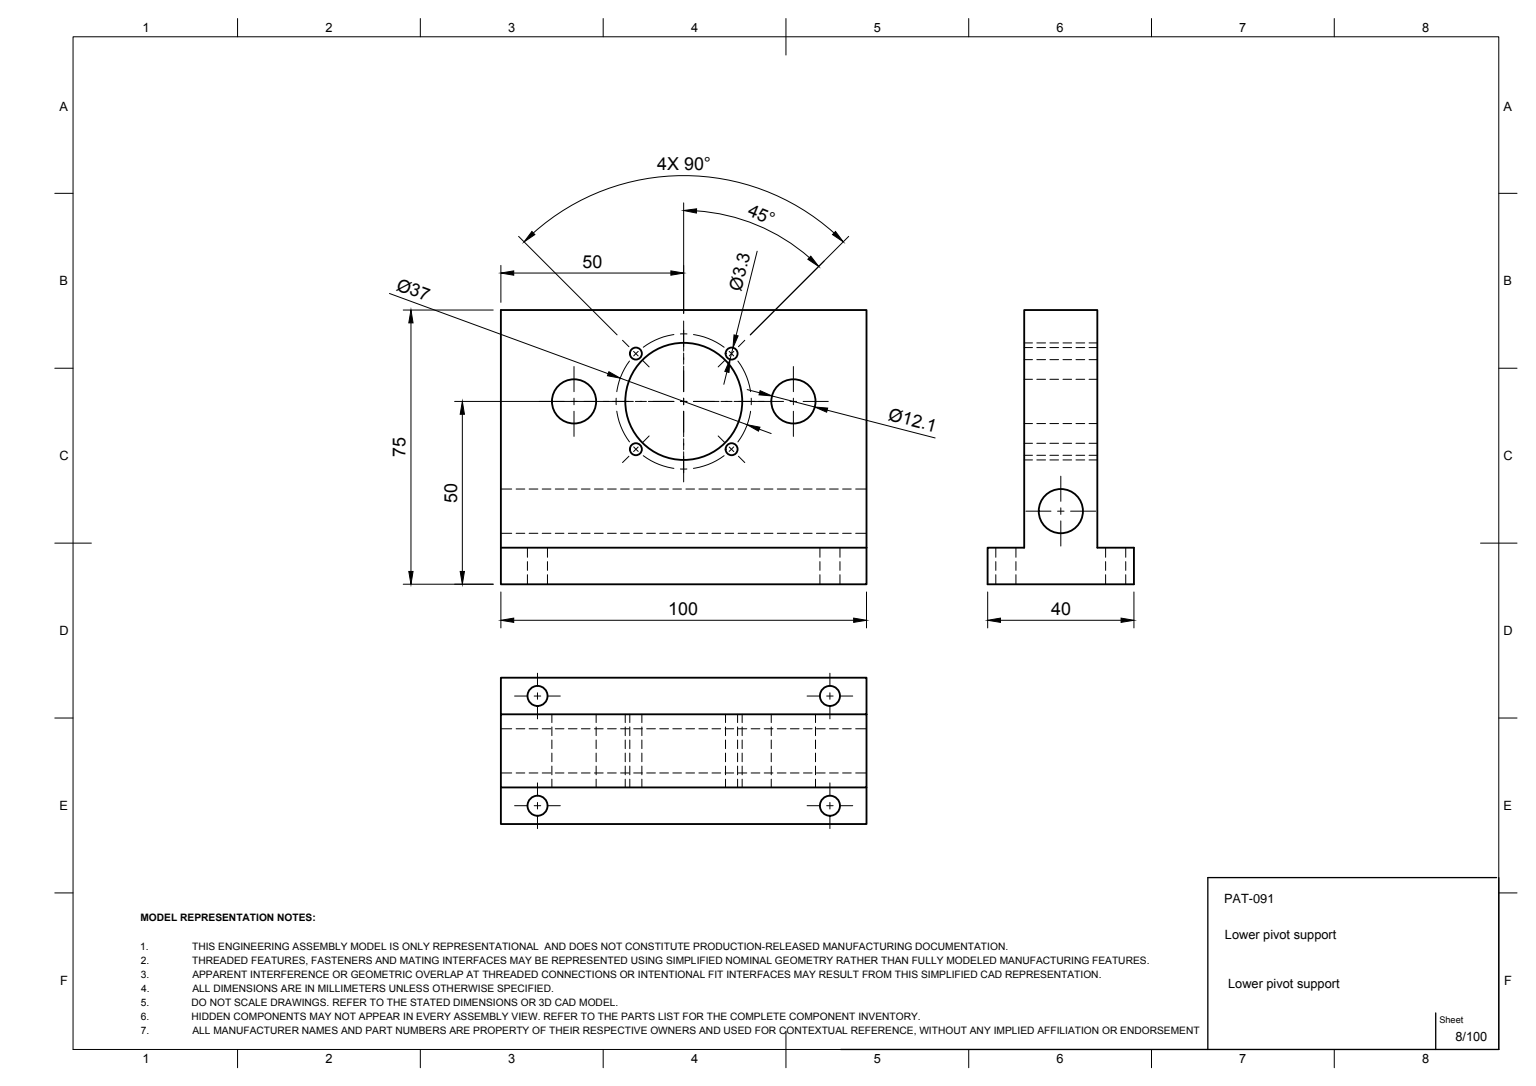
ISO-10303-21;
HEADER;
/* Generated by software containing ST-Developer
 * from STEP Tools, Inc. (www.steptools.com) 
 */

FILE_DESCRIPTION(
/* description */ ('PAT-091'),
/* implementation_level */ '2;1');

FILE_NAME(
/* name */ 'Lower pivot support.step',
/* time_stamp */ '2026-10-27T15:34:44-07:00',
/* author */ (''),
/* organization */ (''),
/* preprocessor_version */ 'ST-DEVELOPER v20.2',
/* originating_system */ 'Autodesk Translation Framework v15.17.0.0',
/* authorisation */ '');

FILE_SCHEMA (('AUTOMOTIVE_DESIGN { 1 0 10303 214 3 1 1 }'));
ENDSEC;

DATA;
#10=MECHANICAL_DESIGN_GEOMETRIC_PRESENTATION_REPRESENTATION('',(#974),#25100);
#754=SHAPE_REPRESENTATION_RELATIONSHIP('SRR','None',#25515,#864);
#864=ADVANCED_BREP_SHAPE_REPRESENTATION('',(#1098),#24985);
#974=STYLED_ITEM('',(#26177),#1098);
#1098=MANIFOLD_SOLID_BREP('Body1',#13251);
#1231=FACE_BOUND('',#2933,.T.);
#1232=FACE_BOUND('',#2934,.T.);
#1233=FACE_BOUND('',#2936,.T.);
#1234=FACE_BOUND('',#2937,.T.);
#1235=FACE_BOUND('',#2941,.T.);
#1236=FACE_BOUND('',#2943,.T.);
#1237=FACE_BOUND('',#2944,.T.);
#1238=FACE_BOUND('',#2945,.T.);
#1239=FACE_BOUND('',#2946,.T.);
#1240=FACE_BOUND('',#2947,.T.);
#1241=FACE_BOUND('',#2948,.T.);
#1242=FACE_BOUND('',#2949,.T.);
#1243=FACE_BOUND('',#2954,.T.);
#1244=FACE_BOUND('',#2955,.T.);
#1245=FACE_BOUND('',#2956,.T.);
#1246=FACE_BOUND('',#2957,.T.);
#1247=FACE_BOUND('',#2958,.T.);
#1248=FACE_BOUND('',#2959,.T.);
#1249=FACE_BOUND('',#2960,.T.);
#1250=FACE_BOUND('',#2962,.T.);
#1251=FACE_BOUND('',#2965,.T.);
#1252=FACE_BOUND('',#2966,.T.);
#1253=FACE_BOUND('',#2967,.T.);
#1254=FACE_BOUND('',#2968,.T.);
#1658=PLANE('',#14660);
#1659=PLANE('',#14661);
#1660=PLANE('',#14662);
#1661=PLANE('',#14663);
#1662=PLANE('',#14664);
#1663=PLANE('',#14666);
#1664=PLANE('',#14675);
#1665=PLANE('',#14676);
#1666=PLANE('',#14677);
#1667=PLANE('',#14678);
#2089=FACE_OUTER_BOUND('',#2923,.T.);
#2090=FACE_OUTER_BOUND('',#2924,.T.);
#2091=FACE_OUTER_BOUND('',#2925,.T.);
#2092=FACE_OUTER_BOUND('',#2926,.T.);
#2093=FACE_OUTER_BOUND('',#2927,.T.);
#2094=FACE_OUTER_BOUND('',#2928,.T.);
#2095=FACE_OUTER_BOUND('',#2929,.T.);
#2096=FACE_OUTER_BOUND('',#2930,.T.);
#2097=FACE_OUTER_BOUND('',#2931,.T.);
#2098=FACE_OUTER_BOUND('',#2932,.T.);
#2099=FACE_OUTER_BOUND('',#2935,.T.);
#2100=FACE_OUTER_BOUND('',#2938,.T.);
#2101=FACE_OUTER_BOUND('',#2939,.T.);
#2102=FACE_OUTER_BOUND('',#2940,.T.);
#2103=FACE_OUTER_BOUND('',#2942,.T.);
#2104=FACE_OUTER_BOUND('',#2950,.T.);
#2105=FACE_OUTER_BOUND('',#2951,.T.);
#2106=FACE_OUTER_BOUND('',#2952,.T.);
#2107=FACE_OUTER_BOUND('',#2953,.T.);
#2108=FACE_OUTER_BOUND('',#2961,.T.);
#2109=FACE_OUTER_BOUND('',#2963,.T.);
#2110=FACE_OUTER_BOUND('',#2964,.T.);
#2923=EDGE_LOOP('',(#9092,#9093,#9094,#9095));
#2924=EDGE_LOOP('',(#9096,#9097,#9098,#9099));
#2925=EDGE_LOOP('',(#9100,#9101,#9102,#9103));
#2926=EDGE_LOOP('',(#9104,#9105,#9106,#9107));
#2927=EDGE_LOOP('',(#9108,#9109,#9110,#9111));
#2928=EDGE_LOOP('',(#9112,#9113,#9114,#9115));
#2929=EDGE_LOOP('',(#9116,#9117,#9118,#9119));
#2930=EDGE_LOOP('',(#9120,#9121,#9122,#9123));
#2931=EDGE_LOOP('',(#9124,#9125,#9126,#9127));
#2932=EDGE_LOOP('',(#9128,#9129,#9130,#9131));
#2933=EDGE_LOOP('',(#9132));
#2934=EDGE_LOOP('',(#9133));
#2935=EDGE_LOOP('',(#9134,#9135,#9136,#9137));
#2936=EDGE_LOOP('',(#9138));
#2937=EDGE_LOOP('',(#9139));
#2938=EDGE_LOOP('',(#9140,#9141,#9142,#9143));
#2939=EDGE_LOOP('',(#9144,#9145,#9146,#9147));
#2940=EDGE_LOOP('',(#9148,#9149,#9150,#9151,#9152,#9153,#9154,#9155));
#2941=EDGE_LOOP('',(#9156));
#2942=EDGE_LOOP('',(#9157,#9158,#9159,#9160));
#2943=EDGE_LOOP('',(#9161));
#2944=EDGE_LOOP('',(#9162));
#2945=EDGE_LOOP('',(#9163));
#2946=EDGE_LOOP('',(#9164));
#2947=EDGE_LOOP('',(#9165));
#2948=EDGE_LOOP('',(#9166));
#2949=EDGE_LOOP('',(#9167));
#2950=EDGE_LOOP('',(#9168,#9169,#9170,#9171));
#2951=EDGE_LOOP('',(#9172,#9173,#9174,#9175));
#2952=EDGE_LOOP('',(#9176,#9177,#9178,#9179));
#2953=EDGE_LOOP('',(#9180,#9181,#9182,#9183));
#2954=EDGE_LOOP('',(#9184));
#2955=EDGE_LOOP('',(#9185));
#2956=EDGE_LOOP('',(#9186));
#2957=EDGE_LOOP('',(#9187));
#2958=EDGE_LOOP('',(#9188));
#2959=EDGE_LOOP('',(#9189));
#2960=EDGE_LOOP('',(#9190));
#2961=EDGE_LOOP('',(#9191,#9192,#9193,#9194,#9195,#9196,#9197,#9198));
#2962=EDGE_LOOP('',(#9199));
#2963=EDGE_LOOP('',(#9200,#9201,#9202,#9203));
#2964=EDGE_LOOP('',(#9204,#9205,#9206,#9207));
#2965=EDGE_LOOP('',(#9208));
#2966=EDGE_LOOP('',(#9209));
#2967=EDGE_LOOP('',(#9210));
#2968=EDGE_LOOP('',(#9211));
#4168=LINE('',#21110,#4908);
#4169=LINE('',#21116,#4909);
#4170=LINE('',#21122,#4910);
#4171=LINE('',#21128,#4911);
#4172=LINE('',#21134,#4912);
#4173=LINE('',#21140,#4913);
#4174=LINE('',#21146,#4914);
#4175=LINE('',#21152,#4915);
#4176=LINE('',#21158,#4916);
#4177=LINE('',#21163,#4917);
#4178=LINE('',#21165,#4918);
#4179=LINE('',#21167,#4919);
#4180=LINE('',#21168,#4920);
#4181=LINE('',#21172,#4921);
#4182=LINE('',#21174,#4922);
#4183=LINE('',#21176,#4923);
#4184=LINE('',#21177,#4924);
#4185=LINE('',#21181,#4925);
#4186=LINE('',#21182,#4926);
#4187=LINE('',#21183,#4927);
#4188=LINE('',#21187,#4928);
#4189=LINE('',#21188,#4929);
#4190=LINE('',#21189,#4930);
#4191=LINE('',#21192,#4931);
#4192=LINE('',#21194,#4932);
#4193=LINE('',#21195,#4933);
#4194=LINE('',#21196,#4934);
#4195=LINE('',#21201,#4935);
#4196=LINE('',#21202,#4936);
#4197=LINE('',#21210,#4937);
#4198=LINE('',#21213,#4938);
#4199=LINE('',#21217,#4939);
#4200=LINE('',#21221,#4940);
#4201=LINE('',#21222,#4941);
#4202=LINE('',#21224,#4942);
#4203=LINE('',#21225,#4943);
#4908=VECTOR('',#16612,0.165);
#4909=VECTOR('',#16619,0.165);
#4910=VECTOR('',#16626,0.165);
#4911=VECTOR('',#16633,0.165);
#4912=VECTOR('',#16640,1.6);
#4913=VECTOR('',#16647,0.275);
#4914=VECTOR('',#16654,0.275);
#4915=VECTOR('',#16661,0.275);
#4916=VECTOR('',#16668,0.275);
#4917=VECTOR('',#16673,1.);
#4918=VECTOR('',#16674,1.);
#4919=VECTOR('',#16675,1.);
#4920=VECTOR('',#16676,1.);
#4921=VECTOR('',#16679,1.);
#4922=VECTOR('',#16680,1.);
#4923=VECTOR('',#16681,1.);
#4924=VECTOR('',#16682,1.);
#4925=VECTOR('',#16685,1.);
#4926=VECTOR('',#16686,1.);
#4927=VECTOR('',#16687,1.);
#4928=VECTOR('',#16690,1.);
#4929=VECTOR('',#16691,1.);
#4930=VECTOR('',#16692,1.);
#4931=VECTOR('',#16695,1.);
#4932=VECTOR('',#16696,1.);
#4933=VECTOR('',#16697,1.);
#4934=VECTOR('',#16698,1.);
#4935=VECTOR('',#16703,1.);
#4936=VECTOR('',#16704,1.);
#4937=VECTOR('',#16713,0.605);
#4938=VECTOR('',#16716,0.605);
#4939=VECTOR('',#16721,0.605);
#4940=VECTOR('',#16726,1.);
#4941=VECTOR('',#16727,1.);
#4942=VECTOR('',#16730,1.);
#4943=VECTOR('',#16731,1.);
#5620=CIRCLE('',#14634,0.165);
#5621=CIRCLE('',#14635,0.165);
#5622=CIRCLE('',#14637,0.165);
#5623=CIRCLE('',#14638,0.165);
#5624=CIRCLE('',#14640,0.165);
#5625=CIRCLE('',#14641,0.165);
#5626=CIRCLE('',#14643,0.165);
#5627=CIRCLE('',#14644,0.165);
#5628=CIRCLE('',#14646,1.6);
#5629=CIRCLE('',#14647,1.6);
#5630=CIRCLE('',#14649,0.275);
#5631=CIRCLE('',#14650,0.275);
#5632=CIRCLE('',#14652,0.275);
#5633=CIRCLE('',#14653,0.275);
#5634=CIRCLE('',#14655,0.275);
#5635=CIRCLE('',#14656,0.275);
#5636=CIRCLE('',#14658,0.275);
#5637=CIRCLE('',#14659,0.275);
#5638=CIRCLE('',#14665,0.605);
#5639=CIRCLE('',#14667,0.605);
#5640=CIRCLE('',#14668,0.605);
#5641=CIRCLE('',#14670,0.605);
#5642=CIRCLE('',#14672,0.605);
#5643=CIRCLE('',#14674,0.605);
#6423=VERTEX_POINT('',#21107);
#6424=VERTEX_POINT('',#21109);
#6425=VERTEX_POINT('',#21113);
#6426=VERTEX_POINT('',#21115);
#6427=VERTEX_POINT('',#21119);
#6428=VERTEX_POINT('',#21121);
#6429=VERTEX_POINT('',#21125);
#6430=VERTEX_POINT('',#21127);
#6431=VERTEX_POINT('',#21131);
#6432=VERTEX_POINT('',#21133);
#6433=VERTEX_POINT('',#21137);
#6434=VERTEX_POINT('',#21139);
#6435=VERTEX_POINT('',#21143);
#6436=VERTEX_POINT('',#21145);
#6437=VERTEX_POINT('',#21149);
#6438=VERTEX_POINT('',#21151);
#6439=VERTEX_POINT('',#21155);
#6440=VERTEX_POINT('',#21157);
#6441=VERTEX_POINT('',#21161);
#6442=VERTEX_POINT('',#21162);
#6443=VERTEX_POINT('',#21164);
#6444=VERTEX_POINT('',#21166);
#6445=VERTEX_POINT('',#21170);
#6446=VERTEX_POINT('',#21171);
#6447=VERTEX_POINT('',#21173);
#6448=VERTEX_POINT('',#21175);
#6449=VERTEX_POINT('',#21179);
#6450=VERTEX_POINT('',#21180);
#6451=VERTEX_POINT('',#21185);
#6452=VERTEX_POINT('',#21186);
#6453=VERTEX_POINT('',#21191);
#6454=VERTEX_POINT('',#21193);
#6455=VERTEX_POINT('',#21197);
#6456=VERTEX_POINT('',#21200);
#6457=VERTEX_POINT('',#21203);
#6458=VERTEX_POINT('',#21205);
#6459=VERTEX_POINT('',#21208);
#6460=VERTEX_POINT('',#21212);
#6461=VERTEX_POINT('',#21216);
#6462=VERTEX_POINT('',#21220);
#7481=EDGE_CURVE('',#6423,#6423,#5620,.T.);
#7482=EDGE_CURVE('',#6423,#6424,#4168,.T.);
#7483=EDGE_CURVE('',#6424,#6424,#5621,.T.);
#7484=EDGE_CURVE('',#6425,#6425,#5622,.T.);
#7485=EDGE_CURVE('',#6425,#6426,#4169,.T.);
#7486=EDGE_CURVE('',#6426,#6426,#5623,.T.);
#7487=EDGE_CURVE('',#6427,#6427,#5624,.T.);
#7488=EDGE_CURVE('',#6427,#6428,#4170,.T.);
#7489=EDGE_CURVE('',#6428,#6428,#5625,.T.);
#7490=EDGE_CURVE('',#6429,#6429,#5626,.T.);
#7491=EDGE_CURVE('',#6429,#6430,#4171,.T.);
#7492=EDGE_CURVE('',#6430,#6430,#5627,.T.);
#7493=EDGE_CURVE('',#6431,#6431,#5628,.T.);
#7494=EDGE_CURVE('',#6431,#6432,#4172,.T.);
#7495=EDGE_CURVE('',#6432,#6432,#5629,.T.);
#7496=EDGE_CURVE('',#6433,#6433,#5630,.T.);
#7497=EDGE_CURVE('',#6433,#6434,#4173,.T.);
#7498=EDGE_CURVE('',#6434,#6434,#5631,.T.);
#7499=EDGE_CURVE('',#6435,#6435,#5632,.T.);
#7500=EDGE_CURVE('',#6435,#6436,#4174,.T.);
#7501=EDGE_CURVE('',#6436,#6436,#5633,.T.);
#7502=EDGE_CURVE('',#6437,#6437,#5634,.T.);
#7503=EDGE_CURVE('',#6437,#6438,#4175,.T.);
#7504=EDGE_CURVE('',#6438,#6438,#5635,.T.);
#7505=EDGE_CURVE('',#6439,#6439,#5636,.T.);
#7506=EDGE_CURVE('',#6439,#6440,#4176,.T.);
#7507=EDGE_CURVE('',#6440,#6440,#5637,.T.);
#7508=EDGE_CURVE('',#6441,#6442,#4177,.T.);
#7509=EDGE_CURVE('',#6441,#6443,#4178,.T.);
#7510=EDGE_CURVE('',#6443,#6444,#4179,.T.);
#7511=EDGE_CURVE('',#6444,#6442,#4180,.T.);
#7512=EDGE_CURVE('',#6445,#6446,#4181,.T.);
#7513=EDGE_CURVE('',#6445,#6447,#4182,.T.);
#7514=EDGE_CURVE('',#6447,#6448,#4183,.T.);
#7515=EDGE_CURVE('',#6448,#6446,#4184,.T.);
#7516=EDGE_CURVE('',#6449,#6450,#4185,.T.);
#7517=EDGE_CURVE('',#6450,#6448,#4186,.T.);
#7518=EDGE_CURVE('',#6449,#6447,#4187,.T.);
#7519=EDGE_CURVE('',#6451,#6452,#4188,.T.);
#7520=EDGE_CURVE('',#6452,#6444,#4189,.T.);
#7521=EDGE_CURVE('',#6451,#6443,#4190,.T.);
#7522=EDGE_CURVE('',#6441,#6453,#4191,.T.);
#7523=EDGE_CURVE('',#6454,#6453,#4192,.T.);
#7524=EDGE_CURVE('',#6446,#6454,#4193,.T.);
#7525=EDGE_CURVE('',#6450,#6451,#4194,.T.);
#7526=EDGE_CURVE('',#6455,#6455,#5638,.T.);
#7527=EDGE_CURVE('',#6442,#6456,#4195,.T.);
#7528=EDGE_CURVE('',#6453,#6456,#4196,.T.);
#7529=EDGE_CURVE('',#6457,#6457,#5639,.T.);
#7530=EDGE_CURVE('',#6458,#6458,#5640,.T.);
#7531=EDGE_CURVE('',#6459,#6459,#5641,.T.);
#7532=EDGE_CURVE('',#6459,#6455,#4197,.T.);
#7533=EDGE_CURVE('',#6457,#6460,#4198,.T.);
#7534=EDGE_CURVE('',#6460,#6460,#5642,.T.);
#7535=EDGE_CURVE('',#6458,#6461,#4199,.T.);
#7536=EDGE_CURVE('',#6461,#6461,#5643,.T.);
#7537=EDGE_CURVE('',#6462,#6454,#4200,.T.);
#7538=EDGE_CURVE('',#6445,#6462,#4201,.T.);
#7539=EDGE_CURVE('',#6456,#6462,#4202,.T.);
#7540=EDGE_CURVE('',#6452,#6449,#4203,.T.);
#9092=ORIENTED_EDGE('',*,*,#7481,.F.);
#9093=ORIENTED_EDGE('',*,*,#7482,.T.);
#9094=ORIENTED_EDGE('',*,*,#7483,.F.);
#9095=ORIENTED_EDGE('',*,*,#7482,.F.);
#9096=ORIENTED_EDGE('',*,*,#7484,.F.);
#9097=ORIENTED_EDGE('',*,*,#7485,.T.);
#9098=ORIENTED_EDGE('',*,*,#7486,.F.);
#9099=ORIENTED_EDGE('',*,*,#7485,.F.);
#9100=ORIENTED_EDGE('',*,*,#7487,.F.);
#9101=ORIENTED_EDGE('',*,*,#7488,.T.);
#9102=ORIENTED_EDGE('',*,*,#7489,.F.);
#9103=ORIENTED_EDGE('',*,*,#7488,.F.);
#9104=ORIENTED_EDGE('',*,*,#7490,.F.);
#9105=ORIENTED_EDGE('',*,*,#7491,.T.);
#9106=ORIENTED_EDGE('',*,*,#7492,.F.);
#9107=ORIENTED_EDGE('',*,*,#7491,.F.);
#9108=ORIENTED_EDGE('',*,*,#7493,.F.);
#9109=ORIENTED_EDGE('',*,*,#7494,.T.);
#9110=ORIENTED_EDGE('',*,*,#7495,.F.);
#9111=ORIENTED_EDGE('',*,*,#7494,.F.);
#9112=ORIENTED_EDGE('',*,*,#7496,.F.);
#9113=ORIENTED_EDGE('',*,*,#7497,.T.);
#9114=ORIENTED_EDGE('',*,*,#7498,.F.);
#9115=ORIENTED_EDGE('',*,*,#7497,.F.);
#9116=ORIENTED_EDGE('',*,*,#7499,.F.);
#9117=ORIENTED_EDGE('',*,*,#7500,.T.);
#9118=ORIENTED_EDGE('',*,*,#7501,.F.);
#9119=ORIENTED_EDGE('',*,*,#7500,.F.);
#9120=ORIENTED_EDGE('',*,*,#7502,.F.);
#9121=ORIENTED_EDGE('',*,*,#7503,.T.);
#9122=ORIENTED_EDGE('',*,*,#7504,.F.);
#9123=ORIENTED_EDGE('',*,*,#7503,.F.);
#9124=ORIENTED_EDGE('',*,*,#7505,.F.);
#9125=ORIENTED_EDGE('',*,*,#7506,.T.);
#9126=ORIENTED_EDGE('',*,*,#7507,.F.);
#9127=ORIENTED_EDGE('',*,*,#7506,.F.);
#9128=ORIENTED_EDGE('',*,*,#7508,.F.);
#9129=ORIENTED_EDGE('',*,*,#7509,.T.);
#9130=ORIENTED_EDGE('',*,*,#7510,.T.);
#9131=ORIENTED_EDGE('',*,*,#7511,.T.);
#9132=ORIENTED_EDGE('',*,*,#7501,.T.);
#9133=ORIENTED_EDGE('',*,*,#7504,.T.);
#9134=ORIENTED_EDGE('',*,*,#7512,.F.);
#9135=ORIENTED_EDGE('',*,*,#7513,.T.);
#9136=ORIENTED_EDGE('',*,*,#7514,.T.);
#9137=ORIENTED_EDGE('',*,*,#7515,.T.);
#9138=ORIENTED_EDGE('',*,*,#7498,.T.);
#9139=ORIENTED_EDGE('',*,*,#7507,.T.);
#9140=ORIENTED_EDGE('',*,*,#7516,.T.);
#9141=ORIENTED_EDGE('',*,*,#7517,.T.);
#9142=ORIENTED_EDGE('',*,*,#7514,.F.);
#9143=ORIENTED_EDGE('',*,*,#7518,.F.);
#9144=ORIENTED_EDGE('',*,*,#7519,.T.);
#9145=ORIENTED_EDGE('',*,*,#7520,.T.);
#9146=ORIENTED_EDGE('',*,*,#7510,.F.);
#9147=ORIENTED_EDGE('',*,*,#7521,.F.);
#9148=ORIENTED_EDGE('',*,*,#7522,.T.);
#9149=ORIENTED_EDGE('',*,*,#7523,.F.);
#9150=ORIENTED_EDGE('',*,*,#7524,.F.);
#9151=ORIENTED_EDGE('',*,*,#7515,.F.);
#9152=ORIENTED_EDGE('',*,*,#7517,.F.);
#9153=ORIENTED_EDGE('',*,*,#7525,.T.);
#9154=ORIENTED_EDGE('',*,*,#7521,.T.);
#9155=ORIENTED_EDGE('',*,*,#7509,.F.);
#9156=ORIENTED_EDGE('',*,*,#7526,.T.);
#9157=ORIENTED_EDGE('',*,*,#7508,.T.);
#9158=ORIENTED_EDGE('',*,*,#7527,.T.);
#9159=ORIENTED_EDGE('',*,*,#7528,.F.);
#9160=ORIENTED_EDGE('',*,*,#7522,.F.);
#9161=ORIENTED_EDGE('',*,*,#7529,.T.);
#9162=ORIENTED_EDGE('',*,*,#7530,.T.);
#9163=ORIENTED_EDGE('',*,*,#7493,.T.);
#9164=ORIENTED_EDGE('',*,*,#7490,.T.);
#9165=ORIENTED_EDGE('',*,*,#7487,.T.);
#9166=ORIENTED_EDGE('',*,*,#7484,.T.);
#9167=ORIENTED_EDGE('',*,*,#7481,.T.);
#9168=ORIENTED_EDGE('',*,*,#7531,.F.);
#9169=ORIENTED_EDGE('',*,*,#7532,.T.);
#9170=ORIENTED_EDGE('',*,*,#7526,.F.);
#9171=ORIENTED_EDGE('',*,*,#7532,.F.);
#9172=ORIENTED_EDGE('',*,*,#7529,.F.);
#9173=ORIENTED_EDGE('',*,*,#7533,.T.);
#9174=ORIENTED_EDGE('',*,*,#7534,.F.);
#9175=ORIENTED_EDGE('',*,*,#7533,.F.);
#9176=ORIENTED_EDGE('',*,*,#7530,.F.);
#9177=ORIENTED_EDGE('',*,*,#7535,.T.);
#9178=ORIENTED_EDGE('',*,*,#7536,.F.);
#9179=ORIENTED_EDGE('',*,*,#7535,.F.);
#9180=ORIENTED_EDGE('',*,*,#7512,.T.);
#9181=ORIENTED_EDGE('',*,*,#7524,.T.);
#9182=ORIENTED_EDGE('',*,*,#7537,.F.);
#9183=ORIENTED_EDGE('',*,*,#7538,.F.);
#9184=ORIENTED_EDGE('',*,*,#7536,.T.);
#9185=ORIENTED_EDGE('',*,*,#7534,.T.);
#9186=ORIENTED_EDGE('',*,*,#7495,.T.);
#9187=ORIENTED_EDGE('',*,*,#7492,.T.);
#9188=ORIENTED_EDGE('',*,*,#7489,.T.);
#9189=ORIENTED_EDGE('',*,*,#7486,.T.);
#9190=ORIENTED_EDGE('',*,*,#7483,.T.);
#9191=ORIENTED_EDGE('',*,*,#7538,.T.);
#9192=ORIENTED_EDGE('',*,*,#7539,.F.);
#9193=ORIENTED_EDGE('',*,*,#7527,.F.);
#9194=ORIENTED_EDGE('',*,*,#7511,.F.);
#9195=ORIENTED_EDGE('',*,*,#7520,.F.);
#9196=ORIENTED_EDGE('',*,*,#7540,.T.);
#9197=ORIENTED_EDGE('',*,*,#7518,.T.);
#9198=ORIENTED_EDGE('',*,*,#7513,.F.);
#9199=ORIENTED_EDGE('',*,*,#7531,.T.);
#9200=ORIENTED_EDGE('',*,*,#7528,.T.);
#9201=ORIENTED_EDGE('',*,*,#7539,.T.);
#9202=ORIENTED_EDGE('',*,*,#7537,.T.);
#9203=ORIENTED_EDGE('',*,*,#7523,.T.);
#9204=ORIENTED_EDGE('',*,*,#7525,.F.);
#9205=ORIENTED_EDGE('',*,*,#7516,.F.);
#9206=ORIENTED_EDGE('',*,*,#7540,.F.);
#9207=ORIENTED_EDGE('',*,*,#7519,.F.);
#9208=ORIENTED_EDGE('',*,*,#7496,.T.);
#9209=ORIENTED_EDGE('',*,*,#7499,.T.);
#9210=ORIENTED_EDGE('',*,*,#7502,.T.);
#9211=ORIENTED_EDGE('',*,*,#7505,.T.);
#12082=CYLINDRICAL_SURFACE('',#14633,0.165);
#12083=CYLINDRICAL_SURFACE('',#14636,0.165);
#12084=CYLINDRICAL_SURFACE('',#14639,0.165);
#12085=CYLINDRICAL_SURFACE('',#14642,0.165);
#12086=CYLINDRICAL_SURFACE('',#14645,1.6);
#12087=CYLINDRICAL_SURFACE('',#14648,0.275);
#12088=CYLINDRICAL_SURFACE('',#14651,0.275);
#12089=CYLINDRICAL_SURFACE('',#14654,0.275);
#12090=CYLINDRICAL_SURFACE('',#14657,0.275);
#12091=CYLINDRICAL_SURFACE('',#14669,0.605);
#12092=CYLINDRICAL_SURFACE('',#14671,0.605);
#12093=CYLINDRICAL_SURFACE('',#14673,0.605);
#12456=ADVANCED_FACE('',(#2089),#12082,.F.);
#12457=ADVANCED_FACE('',(#2090),#12083,.F.);
#12458=ADVANCED_FACE('',(#2091),#12084,.F.);
#12459=ADVANCED_FACE('',(#2092),#12085,.F.);
#12460=ADVANCED_FACE('',(#2093),#12086,.F.);
#12461=ADVANCED_FACE('',(#2094),#12087,.F.);
#12462=ADVANCED_FACE('',(#2095),#12088,.F.);
#12463=ADVANCED_FACE('',(#2096),#12089,.F.);
#12464=ADVANCED_FACE('',(#2097),#12090,.F.);
#12465=ADVANCED_FACE('',(#2098,#1231,#1232),#1658,.T.);
#12466=ADVANCED_FACE('',(#2099,#1233,#1234),#1659,.T.);
#12467=ADVANCED_FACE('',(#2100),#1660,.T.);
#12468=ADVANCED_FACE('',(#2101),#1661,.T.);
#12469=ADVANCED_FACE('',(#2102,#1235),#1662,.T.);
#12470=ADVANCED_FACE('',(#2103,#1236,#1237,#1238,#1239,#1240,#1241,#1242),
#1663,.T.);
#12471=ADVANCED_FACE('',(#2104),#12091,.F.);
#12472=ADVANCED_FACE('',(#2105),#12092,.F.);
#12473=ADVANCED_FACE('',(#2106),#12093,.F.);
#12474=ADVANCED_FACE('',(#2107,#1243,#1244,#1245,#1246,#1247,#1248,#1249),
#1664,.T.);
#12475=ADVANCED_FACE('',(#2108,#1250),#1665,.T.);
#12476=ADVANCED_FACE('',(#2109),#1666,.T.);
#12477=ADVANCED_FACE('',(#2110,#1251,#1252,#1253,#1254),#1667,.F.);
#13251=CLOSED_SHELL('',(#12456,#12457,#12458,#12459,#12460,#12461,#12462,
#12463,#12464,#12465,#12466,#12467,#12468,#12469,#12470,#12471,#12472,#12473,
#12474,#12475,#12476,#12477));
#14632=AXIS2_PLACEMENT_3D('',#21105,#16606,#16607);
#14633=AXIS2_PLACEMENT_3D('',#21106,#16608,#16609);
#14634=AXIS2_PLACEMENT_3D('',#21108,#16610,#16611);
#14635=AXIS2_PLACEMENT_3D('',#21111,#16613,#16614);
#14636=AXIS2_PLACEMENT_3D('',#21112,#16615,#16616);
#14637=AXIS2_PLACEMENT_3D('',#21114,#16617,#16618);
#14638=AXIS2_PLACEMENT_3D('',#21117,#16620,#16621);
#14639=AXIS2_PLACEMENT_3D('',#21118,#16622,#16623);
#14640=AXIS2_PLACEMENT_3D('',#21120,#16624,#16625);
#14641=AXIS2_PLACEMENT_3D('',#21123,#16627,#16628);
#14642=AXIS2_PLACEMENT_3D('',#21124,#16629,#16630);
#14643=AXIS2_PLACEMENT_3D('',#21126,#16631,#16632);
#14644=AXIS2_PLACEMENT_3D('',#21129,#16634,#16635);
#14645=AXIS2_PLACEMENT_3D('',#21130,#16636,#16637);
#14646=AXIS2_PLACEMENT_3D('',#21132,#16638,#16639);
#14647=AXIS2_PLACEMENT_3D('',#21135,#16641,#16642);
#14648=AXIS2_PLACEMENT_3D('',#21136,#16643,#16644);
#14649=AXIS2_PLACEMENT_3D('',#21138,#16645,#16646);
#14650=AXIS2_PLACEMENT_3D('',#21141,#16648,#16649);
#14651=AXIS2_PLACEMENT_3D('',#21142,#16650,#16651);
#14652=AXIS2_PLACEMENT_3D('',#21144,#16652,#16653);
#14653=AXIS2_PLACEMENT_3D('',#21147,#16655,#16656);
#14654=AXIS2_PLACEMENT_3D('',#21148,#16657,#16658);
#14655=AXIS2_PLACEMENT_3D('',#21150,#16659,#16660);
#14656=AXIS2_PLACEMENT_3D('',#21153,#16662,#16663);
#14657=AXIS2_PLACEMENT_3D('',#21154,#16664,#16665);
#14658=AXIS2_PLACEMENT_3D('',#21156,#16666,#16667);
#14659=AXIS2_PLACEMENT_3D('',#21159,#16669,#16670);
#14660=AXIS2_PLACEMENT_3D('',#21160,#16671,#16672);
#14661=AXIS2_PLACEMENT_3D('',#21169,#16677,#16678);
#14662=AXIS2_PLACEMENT_3D('',#21178,#16683,#16684);
#14663=AXIS2_PLACEMENT_3D('',#21184,#16688,#16689);
#14664=AXIS2_PLACEMENT_3D('',#21190,#16693,#16694);
#14665=AXIS2_PLACEMENT_3D('',#21198,#16699,#16700);
#14666=AXIS2_PLACEMENT_3D('',#21199,#16701,#16702);
#14667=AXIS2_PLACEMENT_3D('',#21204,#16705,#16706);
#14668=AXIS2_PLACEMENT_3D('',#21206,#16707,#16708);
#14669=AXIS2_PLACEMENT_3D('',#21207,#16709,#16710);
#14670=AXIS2_PLACEMENT_3D('',#21209,#16711,#16712);
#14671=AXIS2_PLACEMENT_3D('',#21211,#16714,#16715);
#14672=AXIS2_PLACEMENT_3D('',#21214,#16717,#16718);
#14673=AXIS2_PLACEMENT_3D('',#21215,#16719,#16720);
#14674=AXIS2_PLACEMENT_3D('',#21218,#16722,#16723);
#14675=AXIS2_PLACEMENT_3D('',#21219,#16724,#16725);
#14676=AXIS2_PLACEMENT_3D('',#21223,#16728,#16729);
#14677=AXIS2_PLACEMENT_3D('',#21226,#16732,#16733);
#14678=AXIS2_PLACEMENT_3D('',#21227,#16734,#16735);
#16606=DIRECTION('axis',(0.,0.,1.));
#16607=DIRECTION('refdir',(1.,0.,0.));
#16608=DIRECTION('center_axis',(1.,0.,0.));
#16609=DIRECTION('ref_axis',(0.,0.,-1.));
#16610=DIRECTION('center_axis',(1.,0.,0.));
#16611=DIRECTION('ref_axis',(0.,0.,-1.));
#16612=DIRECTION('',(1.,0.,0.));
#16613=DIRECTION('center_axis',(-1.,0.,0.));
#16614=DIRECTION('ref_axis',(0.,0.,-1.));
#16615=DIRECTION('center_axis',(1.,0.,0.));
#16616=DIRECTION('ref_axis',(0.,0.,-1.));
#16617=DIRECTION('center_axis',(1.,0.,0.));
#16618=DIRECTION('ref_axis',(0.,0.,-1.));
#16619=DIRECTION('',(1.,0.,0.));
#16620=DIRECTION('center_axis',(-1.,0.,0.));
#16621=DIRECTION('ref_axis',(0.,0.,-1.));
#16622=DIRECTION('center_axis',(1.,0.,0.));
#16623=DIRECTION('ref_axis',(0.,0.,-1.));
#16624=DIRECTION('center_axis',(1.,0.,0.));
#16625=DIRECTION('ref_axis',(0.,0.,-1.));
#16626=DIRECTION('',(1.,0.,0.));
#16627=DIRECTION('center_axis',(-1.,0.,0.));
#16628=DIRECTION('ref_axis',(0.,0.,-1.));
#16629=DIRECTION('center_axis',(1.,0.,0.));
#16630=DIRECTION('ref_axis',(0.,0.,-1.));
#16631=DIRECTION('center_axis',(1.,0.,0.));
#16632=DIRECTION('ref_axis',(0.,0.,-1.));
#16633=DIRECTION('',(1.,0.,0.));
#16634=DIRECTION('center_axis',(-1.,0.,0.));
#16635=DIRECTION('ref_axis',(0.,0.,-1.));
#16636=DIRECTION('center_axis',(1.,0.,0.));
#16637=DIRECTION('ref_axis',(0.,0.,-1.));
#16638=DIRECTION('center_axis',(1.,0.,0.));
#16639=DIRECTION('ref_axis',(0.,0.,-1.));
#16640=DIRECTION('',(1.,0.,0.));
#16641=DIRECTION('center_axis',(-1.,0.,0.));
#16642=DIRECTION('ref_axis',(0.,0.,-1.));
#16643=DIRECTION('center_axis',(0.,0.,1.));
#16644=DIRECTION('ref_axis',(1.,0.,0.));
#16645=DIRECTION('center_axis',(0.,0.,1.));
#16646=DIRECTION('ref_axis',(1.,0.,0.));
#16647=DIRECTION('',(0.,0.,1.));
#16648=DIRECTION('center_axis',(0.,0.,-1.));
#16649=DIRECTION('ref_axis',(1.,0.,0.));
#16650=DIRECTION('center_axis',(0.,0.,1.));
#16651=DIRECTION('ref_axis',(1.,0.,0.));
#16652=DIRECTION('center_axis',(0.,0.,1.));
#16653=DIRECTION('ref_axis',(1.,0.,0.));
#16654=DIRECTION('',(0.,0.,1.));
#16655=DIRECTION('center_axis',(0.,0.,-1.));
#16656=DIRECTION('ref_axis',(1.,0.,0.));
#16657=DIRECTION('center_axis',(0.,0.,1.));
#16658=DIRECTION('ref_axis',(1.,0.,0.));
#16659=DIRECTION('center_axis',(0.,0.,1.));
#16660=DIRECTION('ref_axis',(1.,0.,0.));
#16661=DIRECTION('',(0.,0.,1.));
#16662=DIRECTION('center_axis',(0.,0.,-1.));
#16663=DIRECTION('ref_axis',(1.,0.,0.));
#16664=DIRECTION('center_axis',(0.,0.,1.));
#16665=DIRECTION('ref_axis',(1.,0.,0.));
#16666=DIRECTION('center_axis',(0.,0.,1.));
#16667=DIRECTION('ref_axis',(1.,0.,0.));
#16668=DIRECTION('',(0.,0.,1.));
#16669=DIRECTION('center_axis',(0.,0.,-1.));
#16670=DIRECTION('ref_axis',(1.,0.,0.));
#16671=DIRECTION('center_axis',(0.,0.,1.));
#16672=DIRECTION('ref_axis',(1.,0.,0.));
#16673=DIRECTION('',(0.,-1.,0.));
#16674=DIRECTION('',(-1.,0.,0.));
#16675=DIRECTION('',(0.,-1.,0.));
#16676=DIRECTION('',(1.,0.,0.));
#16677=DIRECTION('center_axis',(0.,0.,1.));
#16678=DIRECTION('ref_axis',(1.,0.,0.));
#16679=DIRECTION('',(0.,1.,0.));
#16680=DIRECTION('',(1.,0.,0.));
#16681=DIRECTION('',(0.,1.,0.));
#16682=DIRECTION('',(-1.,0.,0.));
#16683=DIRECTION('center_axis',(1.,0.,0.));
#16684=DIRECTION('ref_axis',(0.,1.,0.));
#16685=DIRECTION('',(0.,1.,0.));
#16686=DIRECTION('',(0.,0.,1.));
#16687=DIRECTION('',(0.,0.,1.));
#16688=DIRECTION('center_axis',(-1.,0.,0.));
#16689=DIRECTION('ref_axis',(0.,-1.,0.));
#16690=DIRECTION('',(0.,-1.,0.));
#16691=DIRECTION('',(0.,0.,1.));
#16692=DIRECTION('',(0.,0.,1.));
#16693=DIRECTION('center_axis',(0.,1.,0.));
#16694=DIRECTION('ref_axis',(-1.,0.,0.));
#16695=DIRECTION('',(0.,0.,1.));
#16696=DIRECTION('',(-1.,0.,0.));
#16697=DIRECTION('',(0.,0.,1.));
#16698=DIRECTION('',(-1.,0.,0.));
#16699=DIRECTION('center_axis',(0.,-1.,0.));
#16700=DIRECTION('ref_axis',(1.,0.,0.));
#16701=DIRECTION('center_axis',(-1.,0.,0.));
#16702=DIRECTION('ref_axis',(0.,-1.,0.));
#16703=DIRECTION('',(0.,0.,1.));
#16704=DIRECTION('',(0.,-1.,0.));
#16705=DIRECTION('center_axis',(1.,0.,0.));
#16706=DIRECTION('ref_axis',(0.,0.,-1.));
#16707=DIRECTION('center_axis',(1.,0.,0.));
#16708=DIRECTION('ref_axis',(0.,0.,-1.));
#16709=DIRECTION('center_axis',(0.,1.,0.));
#16710=DIRECTION('ref_axis',(1.,0.,0.));
#16711=DIRECTION('center_axis',(0.,1.,0.));
#16712=DIRECTION('ref_axis',(1.,0.,0.));
#16713=DIRECTION('',(0.,1.,0.));
#16714=DIRECTION('center_axis',(1.,0.,0.));
#16715=DIRECTION('ref_axis',(0.,0.,-1.));
#16716=DIRECTION('',(1.,0.,0.));
#16717=DIRECTION('center_axis',(-1.,0.,0.));
#16718=DIRECTION('ref_axis',(0.,0.,-1.));
#16719=DIRECTION('center_axis',(1.,0.,0.));
#16720=DIRECTION('ref_axis',(0.,0.,-1.));
#16721=DIRECTION('',(1.,0.,0.));
#16722=DIRECTION('center_axis',(-1.,0.,0.));
#16723=DIRECTION('ref_axis',(0.,0.,-1.));
#16724=DIRECTION('center_axis',(1.,0.,0.));
#16725=DIRECTION('ref_axis',(0.,1.,0.));
#16726=DIRECTION('',(0.,1.,0.));
#16727=DIRECTION('',(0.,0.,1.));
#16728=DIRECTION('center_axis',(0.,-1.,0.));
#16729=DIRECTION('ref_axis',(1.,0.,0.));
#16730=DIRECTION('',(1.,0.,0.));
#16731=DIRECTION('',(1.,0.,0.));
#16732=DIRECTION('center_axis',(0.,0.,1.));
#16733=DIRECTION('ref_axis',(1.,0.,0.));
#16734=DIRECTION('center_axis',(0.,0.,1.));
#16735=DIRECTION('ref_axis',(1.,0.,0.));
#21105=CARTESIAN_POINT('',(0.,0.,0.));
#21106=CARTESIAN_POINT('Origin',(-1.1,-1.30814754519511,4.69185245480489));
#21107=CARTESIAN_POINT('',(-1.,-1.30814754519511,4.85685245480489));
#21108=CARTESIAN_POINT('Origin',(-1.,-1.30814754519511,4.69185245480489));
#21109=CARTESIAN_POINT('',(1.,-1.30814754519511,4.85685245480489));
#21110=CARTESIAN_POINT('',(-1.1,-1.30814754519511,4.85685245480489));
#21111=CARTESIAN_POINT('Origin',(1.,-1.30814754519511,4.69185245480489));
#21112=CARTESIAN_POINT('Origin',(-1.1,-1.30814754519511,7.30814754519511));
#21113=CARTESIAN_POINT('',(-1.,-1.30814754519511,7.47314754519511));
#21114=CARTESIAN_POINT('Origin',(-1.,-1.30814754519511,7.30814754519511));
#21115=CARTESIAN_POINT('',(1.,-1.30814754519511,7.47314754519511));
#21116=CARTESIAN_POINT('',(-1.1,-1.30814754519511,7.47314754519511));
#21117=CARTESIAN_POINT('Origin',(1.,-1.30814754519511,7.30814754519511));
#21118=CARTESIAN_POINT('Origin',(-1.1,1.30814754519511,7.30814754519511));
#21119=CARTESIAN_POINT('',(-1.,1.30814754519511,7.47314754519511));
#21120=CARTESIAN_POINT('Origin',(-1.,1.30814754519511,7.30814754519511));
#21121=CARTESIAN_POINT('',(1.,1.30814754519511,7.47314754519511));
#21122=CARTESIAN_POINT('',(-1.1,1.30814754519511,7.47314754519511));
#21123=CARTESIAN_POINT('Origin',(1.,1.30814754519511,7.30814754519511));
#21124=CARTESIAN_POINT('Origin',(-1.1,1.30814754519511,4.69185245480489));
#21125=CARTESIAN_POINT('',(-1.,1.30814754519511,4.85685245480489));
#21126=CARTESIAN_POINT('Origin',(-1.,1.30814754519511,4.69185245480489));
#21127=CARTESIAN_POINT('',(1.,1.30814754519511,4.85685245480489));
#21128=CARTESIAN_POINT('',(-1.1,1.30814754519511,4.85685245480489));
#21129=CARTESIAN_POINT('Origin',(1.,1.30814754519511,4.69185245480489));
#21130=CARTESIAN_POINT('Origin',(-1.1,0.,6.));
#21131=CARTESIAN_POINT('',(-1.,-1.95943487863576E-16,7.6));
#21132=CARTESIAN_POINT('Origin',(-1.,0.,6.));
#21133=CARTESIAN_POINT('',(1.,1.95943487863576E-16,7.6));
#21134=CARTESIAN_POINT('',(-1.1,-1.95943487863576E-16,7.6));
#21135=CARTESIAN_POINT('Origin',(1.,0.,6.));
#21136=CARTESIAN_POINT('Origin',(1.5,-4.,0.9));
#21137=CARTESIAN_POINT('',(1.225,-4.,1.));
#21138=CARTESIAN_POINT('Origin',(1.5,-4.,1.));
#21139=CARTESIAN_POINT('',(1.225,-4.,2.));
#21140=CARTESIAN_POINT('',(1.225,-4.,0.9));
#21141=CARTESIAN_POINT('Origin',(1.5,-4.,2.));
#21142=CARTESIAN_POINT('Origin',(-1.5,4.,0.9));
#21143=CARTESIAN_POINT('',(-1.775,4.,1.));
#21144=CARTESIAN_POINT('Origin',(-1.5,4.,1.));
#21145=CARTESIAN_POINT('',(-1.775,4.,2.));
#21146=CARTESIAN_POINT('',(-1.775,4.,0.9));
#21147=CARTESIAN_POINT('Origin',(-1.5,4.,2.));
#21148=CARTESIAN_POINT('Origin',(-1.5,-4.,0.9));
#21149=CARTESIAN_POINT('',(-1.775,-4.,1.));
#21150=CARTESIAN_POINT('Origin',(-1.5,-4.,1.));
#21151=CARTESIAN_POINT('',(-1.775,-4.,2.));
#21152=CARTESIAN_POINT('',(-1.775,-4.,0.9));
#21153=CARTESIAN_POINT('Origin',(-1.5,-4.,2.));
#21154=CARTESIAN_POINT('Origin',(1.5,4.,0.9));
#21155=CARTESIAN_POINT('',(1.225,4.,1.));
#21156=CARTESIAN_POINT('Origin',(1.5,4.,1.));
#21157=CARTESIAN_POINT('',(1.225,4.,2.));
#21158=CARTESIAN_POINT('',(1.225,4.,0.9));
#21159=CARTESIAN_POINT('Origin',(1.5,4.,2.));
#21160=CARTESIAN_POINT('Origin',(0.,0.,2.));
#21161=CARTESIAN_POINT('',(-1.,5.,2.));
#21162=CARTESIAN_POINT('',(-1.,-5.,2.));
#21163=CARTESIAN_POINT('',(-1.,2.5,2.));
#21164=CARTESIAN_POINT('',(-2.,5.,2.));
#21165=CARTESIAN_POINT('',(2.,5.,2.));
#21166=CARTESIAN_POINT('',(-2.,-5.,2.));
#21167=CARTESIAN_POINT('',(-2.,5.,2.));
#21168=CARTESIAN_POINT('',(-2.,-5.,2.));
#21169=CARTESIAN_POINT('Origin',(0.,0.,2.));
#21170=CARTESIAN_POINT('',(1.,-5.,2.));
#21171=CARTESIAN_POINT('',(1.,5.,2.));
#21172=CARTESIAN_POINT('',(1.,-2.5,2.));
#21173=CARTESIAN_POINT('',(2.,-5.,2.));
#21174=CARTESIAN_POINT('',(-2.,-5.,2.));
#21175=CARTESIAN_POINT('',(2.,5.,2.));
#21176=CARTESIAN_POINT('',(2.,-5.,2.));
#21177=CARTESIAN_POINT('',(2.,5.,2.));
#21178=CARTESIAN_POINT('Origin',(2.,-5.,1.));
#21179=CARTESIAN_POINT('',(2.,-5.,1.));
#21180=CARTESIAN_POINT('',(2.,5.,1.));
#21181=CARTESIAN_POINT('',(2.,-5.,1.));
#21182=CARTESIAN_POINT('',(2.,5.,1.));
#21183=CARTESIAN_POINT('',(2.,-5.,1.));
#21184=CARTESIAN_POINT('Origin',(-2.,5.,1.));
#21185=CARTESIAN_POINT('',(-2.,5.,1.));
#21186=CARTESIAN_POINT('',(-2.,-5.,1.));
#21187=CARTESIAN_POINT('',(-2.,5.,1.));
#21188=CARTESIAN_POINT('',(-2.,-5.,1.));
#21189=CARTESIAN_POINT('',(-2.,5.,1.));
#21190=CARTESIAN_POINT('Origin',(1.,5.,1.));
#21191=CARTESIAN_POINT('',(-1.,5.,8.5));
#21192=CARTESIAN_POINT('',(-1.,5.,1.));
#21193=CARTESIAN_POINT('',(1.,5.,8.5));
#21194=CARTESIAN_POINT('',(1.,5.,8.5));
#21195=CARTESIAN_POINT('',(1.,5.,1.));
#21196=CARTESIAN_POINT('',(2.,5.,1.));
#21197=CARTESIAN_POINT('',(-0.605,5.,3.));
#21198=CARTESIAN_POINT('Origin',(0.,5.,3.));
#21199=CARTESIAN_POINT('Origin',(-1.,5.,1.));
#21200=CARTESIAN_POINT('',(-1.,-5.,8.5));
#21201=CARTESIAN_POINT('',(-1.,-5.,1.));
#21202=CARTESIAN_POINT('',(-1.,5.,8.5));
#21203=CARTESIAN_POINT('',(-1.,-3.,6.605));
#21204=CARTESIAN_POINT('Origin',(-1.,-3.,6.));
#21205=CARTESIAN_POINT('',(-1.,3.,6.605));
#21206=CARTESIAN_POINT('Origin',(-1.,3.,6.));
#21207=CARTESIAN_POINT('Origin',(0.,-5.1,3.));
#21208=CARTESIAN_POINT('',(-0.605,-5.,3.));
#21209=CARTESIAN_POINT('Origin',(0.,-5.,3.));
#21210=CARTESIAN_POINT('',(-0.605,-5.1,3.));
#21211=CARTESIAN_POINT('Origin',(-1.1,-3.,6.));
#21212=CARTESIAN_POINT('',(1.,-3.,6.605));
#21213=CARTESIAN_POINT('',(-1.1,-3.,6.605));
#21214=CARTESIAN_POINT('Origin',(1.,-3.,6.));
#21215=CARTESIAN_POINT('Origin',(-1.1,3.,6.));
#21216=CARTESIAN_POINT('',(1.,3.,6.605));
#21217=CARTESIAN_POINT('',(-1.1,3.,6.605));
#21218=CARTESIAN_POINT('Origin',(1.,3.,6.));
#21219=CARTESIAN_POINT('Origin',(1.,-5.,1.));
#21220=CARTESIAN_POINT('',(1.,-5.,8.5));
#21221=CARTESIAN_POINT('',(1.,-5.,8.5));
#21222=CARTESIAN_POINT('',(1.,-5.,1.));
#21223=CARTESIAN_POINT('Origin',(-1.,-5.,1.));
#21224=CARTESIAN_POINT('',(-1.,-5.,8.5));
#21225=CARTESIAN_POINT('',(-2.,-5.,1.));
#21226=CARTESIAN_POINT('Origin',(0.,0.,8.5));
#21227=CARTESIAN_POINT('Origin',(0.,0.,1.));
#24864=UNCERTAINTY_MEASURE_WITH_UNIT(LENGTH_MEASURE(0.001),#25101,
'DISTANCE_ACCURACY_VALUE',
'Maximum model space distance between geometric entities at asserted c
onnectivities');
#24979=UNCERTAINTY_MEASURE_WITH_UNIT(LENGTH_MEASURE(0.001),#25101,
'DISTANCE_ACCURACY_VALUE',
'Maximum model space distance between geometric entities at asserted c
onnectivities');
#24985=(
GEOMETRIC_REPRESENTATION_CONTEXT(3)
GLOBAL_UNCERTAINTY_ASSIGNED_CONTEXT((#24864))
GLOBAL_UNIT_ASSIGNED_CONTEXT((#25101,#25103,#25104))
REPRESENTATION_CONTEXT('','3D')
);
#25100=(
GEOMETRIC_REPRESENTATION_CONTEXT(3)
GLOBAL_UNCERTAINTY_ASSIGNED_CONTEXT((#24979))
GLOBAL_UNIT_ASSIGNED_CONTEXT((#25101,#25103,#25104))
REPRESENTATION_CONTEXT('','3D')
);
#25101=(
LENGTH_UNIT()
NAMED_UNIT(*)
SI_UNIT(.CENTI.,.METRE.)
);
#25103=(
NAMED_UNIT(*)
PLANE_ANGLE_UNIT()
SI_UNIT($,.RADIAN.)
);
#25104=(
NAMED_UNIT(*)
SI_UNIT($,.STERADIAN.)
SOLID_ANGLE_UNIT()
);
#25110=SHAPE_DEFINITION_REPRESENTATION(#25230,#25515);
#25230=PRODUCT_DEFINITION_SHAPE('',$,#25636);
#25515=SHAPE_REPRESENTATION('',(#14632),#24985);
#25630=PRODUCT_DEFINITION_CONTEXT('part definition',#25992,'design');
#25636=PRODUCT_DEFINITION('Lower pivot support','Lower pivot support',#25756,
#25630);
#25756=PRODUCT_DEFINITION_FORMATION('',$,#25999);
#25992=APPLICATION_CONTEXT(
'Core Data for Automotive Mechanical Design Process');
#25993=PRODUCT_CONTEXT('part definition',#25992,'mechanical');
#25999=PRODUCT('Lower pivot support','Lower pivot support',
'Lower pivot support',(#25993));
#26171=COLOUR_RGB('Light Blue',0.38,0.62,0.78);
#26172=FILL_AREA_STYLE_COLOUR('',#26171);
#26173=FILL_AREA_STYLE('',(#26172));
#26174=SURFACE_STYLE_FILL_AREA(#26173);
#26175=SURFACE_SIDE_STYLE('',(#26174));
#26176=SURFACE_STYLE_USAGE(.BOTH.,#26175);
#26177=PRESENTATION_STYLE_ASSIGNMENT((#26176));
ENDSEC;
END-ISO-10303-21;
